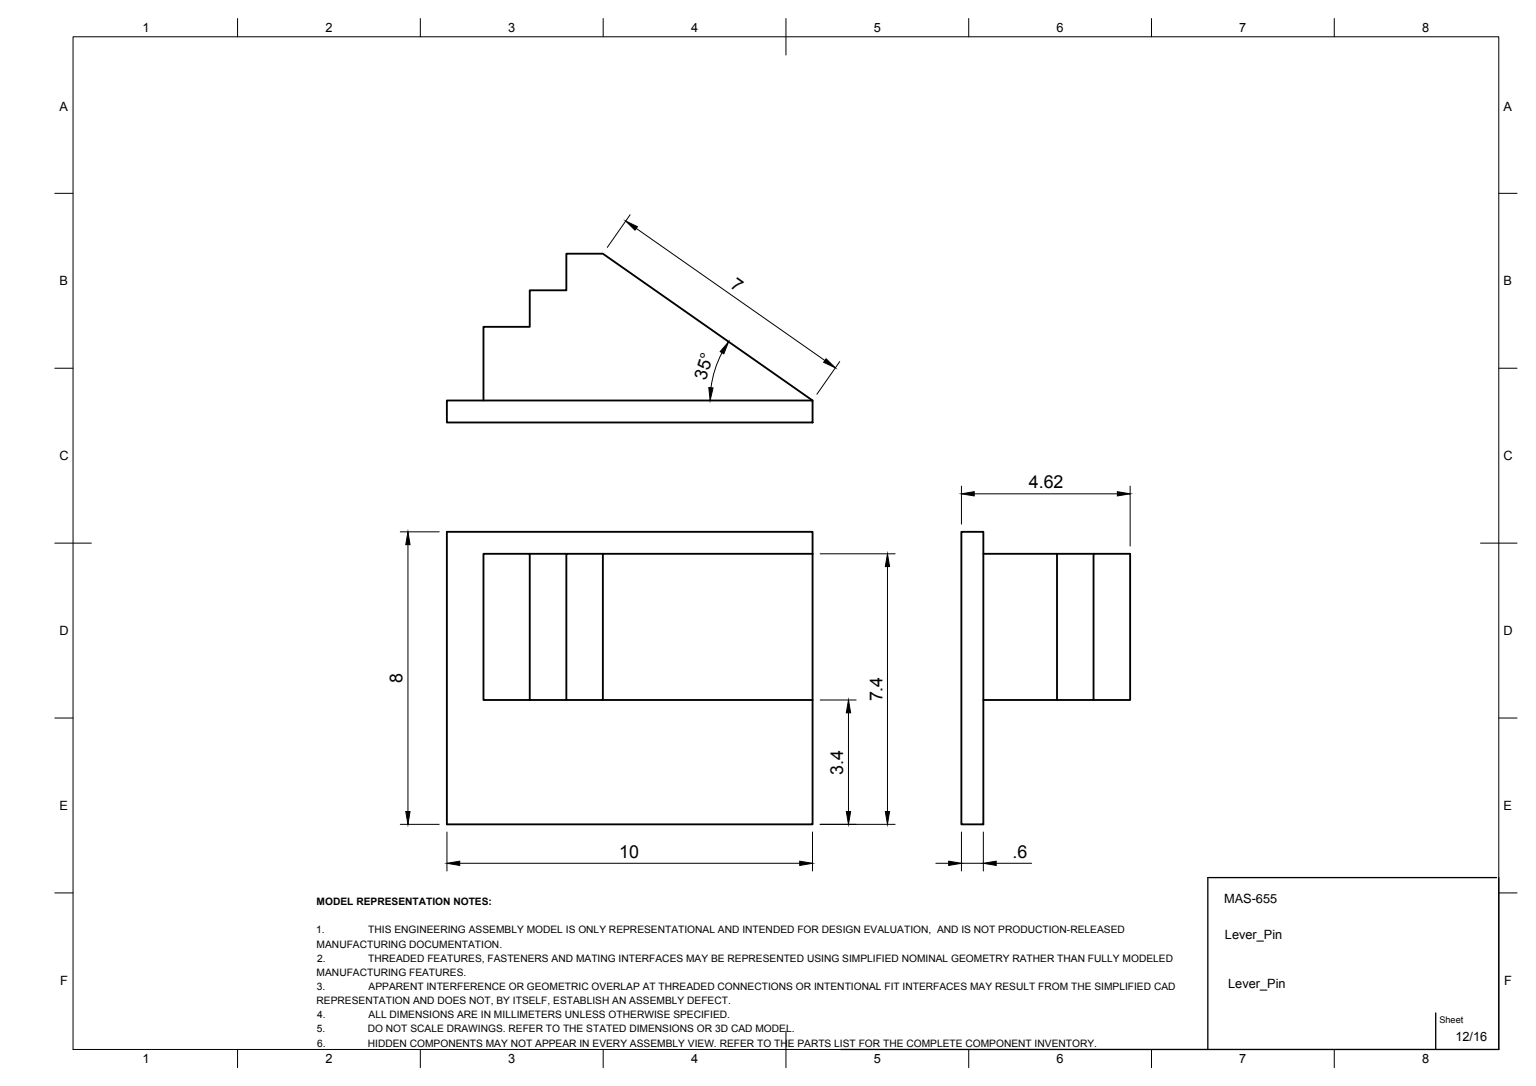
ISO-10303-21;
HEADER;
FILE_DESCRIPTION((''),'2;1');
FILE_NAME('Lever_Pin.step','2026-10-09T11:34:15-07:00',(''),(''),'','','');
FILE_SCHEMA (('AUTOMOTIVE_DESIGN { 1 0 10303 214 3 1 1 }'));
ENDSEC;
DATA;
#10=MECHANICAL_DESIGN_GEOMETRIC_PRESENTATION_REPRESENTATION('',(#644),#117170);
#602=SHAPE_REPRESENTATION_RELATIONSHIP('SRR','None',#117257,#623) ;
#623=ADVANCED_BREP_SHAPE_REPRESENTATION('',(#665),#117165) ;
#644=STYLED_ITEM('',(#117355),#665) ;
#665=MANIFOLD_SOLID_BREP('Body1',#49073) ;
#2840=PLANE('',#54012) ;
#2841=PLANE('',#54013) ;
#2842=PLANE('',#54014) ;
#2843=PLANE('',#54015) ;
#2844=PLANE('',#54016) ;
#2845=PLANE('',#54017) ;
#2846=PLANE('',#54018) ;
#2847=PLANE('',#54019) ;
#2848=PLANE('',#54020) ;
#2849=PLANE('',#54021) ;
#2850=PLANE('',#54022) ;
#2851=PLANE('',#54023) ;
#2852=PLANE('',#54024) ;
#2853=PLANE('',#54025) ;
#2854=PLANE('',#54026) ;
#5713=LINE('',#98676,#8927) ;
#5714=LINE('',#98678,#8928) ;
#5715=LINE('',#98680,#8929) ;
#5716=LINE('',#98681,#8930) ;
#5717=LINE('',#98684,#8931) ;
#5718=LINE('',#98686,#8932) ;
#5719=LINE('',#98687,#8933) ;
#5720=LINE('',#98690,#8934) ;
#5721=LINE('',#98692,#8935) ;
#5722=LINE('',#98693,#8936) ;
#5723=LINE('',#98696,#8937) ;
#5724=LINE('',#98698,#8938) ;
#5725=LINE('',#98699,#8939) ;
#5726=LINE('',#98702,#8940) ;
#5727=LINE('',#98704,#8941) ;
#5728=LINE('',#98705,#8942) ;
#5729=LINE('',#98708,#8943) ;
#5730=LINE('',#98710,#8944) ;
#5731=LINE('',#98711,#8945) ;
#5732=LINE('',#98714,#8946) ;
#5733=LINE('',#98716,#8947) ;
#5734=LINE('',#98717,#8948) ;
#5735=LINE('',#98719,#8949) ;
#5736=LINE('',#98721,#8950) ;
#5737=LINE('',#98725,#8951) ;
#5738=LINE('',#98727,#8952) ;
#5739=LINE('',#98729,#8953) ;
#5740=LINE('',#98730,#8954) ;
#5741=LINE('',#98733,#8955) ;
#5742=LINE('',#98734,#8956) ;
#5743=LINE('',#98736,#8957) ;
#5744=LINE('',#98737,#8958) ;
#5745=LINE('',#98740,#8959) ;
#5746=LINE('',#98742,#8960) ;
#5747=LINE('',#98743,#8961) ;
#5748=LINE('',#98745,#8962) ;
#5749=LINE('',#98746,#8963) ;
#8927=VECTOR('',#67184,10.) ;
#8928=VECTOR('',#67185,10.) ;
#8929=VECTOR('',#67186,10.) ;
#8930=VECTOR('',#67187,10.) ;
#8931=VECTOR('',#67190,10.) ;
#8932=VECTOR('',#67191,10.) ;
#8933=VECTOR('',#67192,10.) ;
#8934=VECTOR('',#67195,10.) ;
#8935=VECTOR('',#67196,10.) ;
#8936=VECTOR('',#67197,10.) ;
#8937=VECTOR('',#67200,10.) ;
#8938=VECTOR('',#67201,10.) ;
#8939=VECTOR('',#67202,10.) ;
#8940=VECTOR('',#67205,10.) ;
#8941=VECTOR('',#67206,10.) ;
#8942=VECTOR('',#67207,10.) ;
#8943=VECTOR('',#67210,10.) ;
#8944=VECTOR('',#67211,10.) ;
#8945=VECTOR('',#67212,10.) ;
#8946=VECTOR('',#67215,10.) ;
#8947=VECTOR('',#67216,10.) ;
#8948=VECTOR('',#67217,10.) ;
#8949=VECTOR('',#67220,10.) ;
#8950=VECTOR('',#67223,10.) ;
#8951=VECTOR('',#67226,10.) ;
#8952=VECTOR('',#67227,10.) ;
#8953=VECTOR('',#67228,10.) ;
#8954=VECTOR('',#67229,10.) ;
#8955=VECTOR('',#67232,10.) ;
#8956=VECTOR('',#67233,10.) ;
#8957=VECTOR('',#67234,10.) ;
#8958=VECTOR('',#67235,10.) ;
#8959=VECTOR('',#67238,10.) ;
#8960=VECTOR('',#67239,10.) ;
#8961=VECTOR('',#67240,10.) ;
#8962=VECTOR('',#67243,10.) ;
#8963=VECTOR('',#67244,10.) ;
#13208=FACE_OUTER_BOUND('',#16391,.T.) ;
#13209=FACE_OUTER_BOUND('',#16392,.T.) ;
#13210=FACE_OUTER_BOUND('',#16393,.T.) ;
#13211=FACE_OUTER_BOUND('',#16394,.T.) ;
#13212=FACE_OUTER_BOUND('',#16395,.T.) ;
#13213=FACE_OUTER_BOUND('',#16396,.T.) ;
#13214=FACE_OUTER_BOUND('',#16397,.T.) ;
#13215=FACE_OUTER_BOUND('',#16398,.T.) ;
#13216=FACE_OUTER_BOUND('',#16399,.T.) ;
#13217=FACE_OUTER_BOUND('',#16400,.T.) ;
#13218=FACE_OUTER_BOUND('',#16401,.T.) ;
#13219=FACE_OUTER_BOUND('',#16402,.T.) ;
#13220=FACE_OUTER_BOUND('',#16403,.T.) ;
#13221=FACE_OUTER_BOUND('',#16404,.T.) ;
#13222=FACE_OUTER_BOUND('',#16405,.T.) ;
#16391=EDGE_LOOP('',(#42608,#42609,#42610,#42611)) ;
#16392=EDGE_LOOP('',(#42612,#42613,#42614,#42615)) ;
#16393=EDGE_LOOP('',(#42616,#42617,#42618,#42619)) ;
#16394=EDGE_LOOP('',(#42620,#42621,#42622,#42623)) ;
#16395=EDGE_LOOP('',(#42624,#42625,#42626,#42627)) ;
#16396=EDGE_LOOP('',(#42628,#42629,#42630,#42631)) ;
#16397=EDGE_LOOP('',(#42632,#42633,#42634,#42635)) ;
#16398=EDGE_LOOP('',(#42636,#42637,#42638,#42639,#42640,#42641,#42642,#42643)) ;
#16399=EDGE_LOOP('',(#42644,#42645,#42646,#42647,#42648,#42649,#42650,#42651)) ;
#16400=EDGE_LOOP('',(#42652,#42653,#42654,#42655)) ;
#16401=EDGE_LOOP('',(#42656,#42657,#42658,#42659,#42660,#42661,#42662,#42663)) ;
#16402=EDGE_LOOP('',(#42664,#42665,#42666,#42667,#42668,#42669)) ;
#16403=EDGE_LOOP('',(#42670,#42671,#42672,#42673)) ;
#16404=EDGE_LOOP('',(#42674,#42675,#42676,#42677)) ;
#16405=EDGE_LOOP('',(#42678,#42679,#42680,#42681)) ;
#22976=VERTEX_POINT('',#98674) ;
#22977=VERTEX_POINT('',#98675) ;
#22978=VERTEX_POINT('',#98677) ;
#22979=VERTEX_POINT('',#98679) ;
#22980=VERTEX_POINT('',#98683) ;
#22981=VERTEX_POINT('',#98685) ;
#22982=VERTEX_POINT('',#98689) ;
#22983=VERTEX_POINT('',#98691) ;
#22984=VERTEX_POINT('',#98695) ;
#22985=VERTEX_POINT('',#98697) ;
#22986=VERTEX_POINT('',#98701) ;
#22987=VERTEX_POINT('',#98703) ;
#22988=VERTEX_POINT('',#98707) ;
#22989=VERTEX_POINT('',#98709) ;
#22990=VERTEX_POINT('',#98713) ;
#22991=VERTEX_POINT('',#98715) ;
#22992=VERTEX_POINT('',#98723) ;
#22993=VERTEX_POINT('',#98724) ;
#22994=VERTEX_POINT('',#98726) ;
#22995=VERTEX_POINT('',#98728) ;
#22996=VERTEX_POINT('',#98732) ;
#22997=VERTEX_POINT('',#98735) ;
#22998=VERTEX_POINT('',#98739) ;
#22999=VERTEX_POINT('',#98741) ;
#29582=EDGE_CURVE('',#22976,#22977,#5713,.T.) ;
#29583=EDGE_CURVE('',#22978,#22977,#5714,.T.) ;
#29584=EDGE_CURVE('',#22979,#22978,#5715,.T.) ;
#29585=EDGE_CURVE('',#22976,#22979,#5716,.T.) ;
#29586=EDGE_CURVE('',#22980,#22976,#5717,.T.) ;
#29587=EDGE_CURVE('',#22981,#22979,#5718,.T.) ;
#29588=EDGE_CURVE('',#22980,#22981,#5719,.T.) ;
#29589=EDGE_CURVE('',#22982,#22980,#5720,.T.) ;
#29590=EDGE_CURVE('',#22983,#22981,#5721,.T.) ;
#29591=EDGE_CURVE('',#22982,#22983,#5722,.T.) ;
#29592=EDGE_CURVE('',#22984,#22982,#5723,.T.) ;
#29593=EDGE_CURVE('',#22985,#22983,#5724,.T.) ;
#29594=EDGE_CURVE('',#22984,#22985,#5725,.T.) ;
#29595=EDGE_CURVE('',#22986,#22984,#5726,.T.) ;
#29596=EDGE_CURVE('',#22987,#22985,#5727,.T.) ;
#29597=EDGE_CURVE('',#22986,#22987,#5728,.T.) ;
#29598=EDGE_CURVE('',#22988,#22986,#5729,.T.) ;
#29599=EDGE_CURVE('',#22989,#22987,#5730,.T.) ;
#29600=EDGE_CURVE('',#22988,#22989,#5731,.T.) ;
#29601=EDGE_CURVE('',#22990,#22988,#5732,.T.) ;
#29602=EDGE_CURVE('',#22991,#22989,#5733,.T.) ;
#29603=EDGE_CURVE('',#22990,#22991,#5734,.T.) ;
#29604=EDGE_CURVE('',#22991,#22978,#5735,.T.) ;
#29605=EDGE_CURVE('',#22977,#22990,#5736,.T.) ;
#29606=EDGE_CURVE('',#22992,#22993,#5737,.T.) ;
#29607=EDGE_CURVE('',#22993,#22994,#5738,.T.) ;
#29608=EDGE_CURVE('',#22995,#22994,#5739,.T.) ;
#29609=EDGE_CURVE('',#22992,#22995,#5740,.T.) ;
#29610=EDGE_CURVE('',#22996,#22990,#5741,.T.) ;
#29611=EDGE_CURVE('',#22996,#22992,#5742,.T.) ;
#29612=EDGE_CURVE('',#22997,#22995,#5743,.T.) ;
#29613=EDGE_CURVE('',#22991,#22997,#5744,.T.) ;
#29614=EDGE_CURVE('',#22998,#22996,#5745,.T.) ;
#29615=EDGE_CURVE('',#22999,#22997,#5746,.T.) ;
#29616=EDGE_CURVE('',#22998,#22999,#5747,.T.) ;
#29617=EDGE_CURVE('',#22993,#22998,#5748,.T.) ;
#29618=EDGE_CURVE('',#22994,#22999,#5749,.T.) ;
#42608=ORIENTED_EDGE('',*,*,#29582,.T.) ;
#42609=ORIENTED_EDGE('',*,*,#29583,.F.) ;
#42610=ORIENTED_EDGE('',*,*,#29584,.F.) ;
#42611=ORIENTED_EDGE('',*,*,#29585,.F.) ;
#42612=ORIENTED_EDGE('',*,*,#29586,.T.) ;
#42613=ORIENTED_EDGE('',*,*,#29585,.T.) ;
#42614=ORIENTED_EDGE('',*,*,#29587,.F.) ;
#42615=ORIENTED_EDGE('',*,*,#29588,.F.) ;
#42616=ORIENTED_EDGE('',*,*,#29589,.T.) ;
#42617=ORIENTED_EDGE('',*,*,#29588,.T.) ;
#42618=ORIENTED_EDGE('',*,*,#29590,.F.) ;
#42619=ORIENTED_EDGE('',*,*,#29591,.F.) ;
#42620=ORIENTED_EDGE('',*,*,#29592,.T.) ;
#42621=ORIENTED_EDGE('',*,*,#29591,.T.) ;
#42622=ORIENTED_EDGE('',*,*,#29593,.F.) ;
#42623=ORIENTED_EDGE('',*,*,#29594,.F.) ;
#42624=ORIENTED_EDGE('',*,*,#29595,.T.) ;
#42625=ORIENTED_EDGE('',*,*,#29594,.T.) ;
#42626=ORIENTED_EDGE('',*,*,#29596,.F.) ;
#42627=ORIENTED_EDGE('',*,*,#29597,.F.) ;
#42628=ORIENTED_EDGE('',*,*,#29598,.T.) ;
#42629=ORIENTED_EDGE('',*,*,#29597,.T.) ;
#42630=ORIENTED_EDGE('',*,*,#29599,.F.) ;
#42631=ORIENTED_EDGE('',*,*,#29600,.F.) ;
#42632=ORIENTED_EDGE('',*,*,#29601,.T.) ;
#42633=ORIENTED_EDGE('',*,*,#29600,.T.) ;
#42634=ORIENTED_EDGE('',*,*,#29602,.F.) ;
#42635=ORIENTED_EDGE('',*,*,#29603,.F.) ;
#42636=ORIENTED_EDGE('',*,*,#29602,.T.) ;
#42637=ORIENTED_EDGE('',*,*,#29599,.T.) ;
#42638=ORIENTED_EDGE('',*,*,#29596,.T.) ;
#42639=ORIENTED_EDGE('',*,*,#29593,.T.) ;
#42640=ORIENTED_EDGE('',*,*,#29590,.T.) ;
#42641=ORIENTED_EDGE('',*,*,#29587,.T.) ;
#42642=ORIENTED_EDGE('',*,*,#29584,.T.) ;
#42643=ORIENTED_EDGE('',*,*,#29604,.F.) ;
#42644=ORIENTED_EDGE('',*,*,#29601,.F.) ;
#42645=ORIENTED_EDGE('',*,*,#29605,.F.) ;
#42646=ORIENTED_EDGE('',*,*,#29582,.F.) ;
#42647=ORIENTED_EDGE('',*,*,#29586,.F.) ;
#42648=ORIENTED_EDGE('',*,*,#29589,.F.) ;
#42649=ORIENTED_EDGE('',*,*,#29592,.F.) ;
#42650=ORIENTED_EDGE('',*,*,#29595,.F.) ;
#42651=ORIENTED_EDGE('',*,*,#29598,.F.) ;
#42652=ORIENTED_EDGE('',*,*,#29606,.T.) ;
#42653=ORIENTED_EDGE('',*,*,#29607,.T.) ;
#42654=ORIENTED_EDGE('',*,*,#29608,.F.) ;
#42655=ORIENTED_EDGE('',*,*,#29609,.F.) ;
#42656=ORIENTED_EDGE('',*,*,#29605,.T.) ;
#42657=ORIENTED_EDGE('',*,*,#29610,.F.) ;
#42658=ORIENTED_EDGE('',*,*,#29611,.T.) ;
#42659=ORIENTED_EDGE('',*,*,#29609,.T.) ;
#42660=ORIENTED_EDGE('',*,*,#29612,.F.) ;
#42661=ORIENTED_EDGE('',*,*,#29613,.F.) ;
#42662=ORIENTED_EDGE('',*,*,#29604,.T.) ;
#42663=ORIENTED_EDGE('',*,*,#29583,.T.) ;
#42664=ORIENTED_EDGE('',*,*,#29614,.T.) ;
#42665=ORIENTED_EDGE('',*,*,#29610,.T.) ;
#42666=ORIENTED_EDGE('',*,*,#29603,.T.) ;
#42667=ORIENTED_EDGE('',*,*,#29613,.T.) ;
#42668=ORIENTED_EDGE('',*,*,#29615,.F.) ;
#42669=ORIENTED_EDGE('',*,*,#29616,.F.) ;
#42670=ORIENTED_EDGE('',*,*,#29617,.T.) ;
#42671=ORIENTED_EDGE('',*,*,#29616,.T.) ;
#42672=ORIENTED_EDGE('',*,*,#29618,.F.) ;
#42673=ORIENTED_EDGE('',*,*,#29607,.F.) ;
#42674=ORIENTED_EDGE('',*,*,#29618,.T.) ;
#42675=ORIENTED_EDGE('',*,*,#29615,.T.) ;
#42676=ORIENTED_EDGE('',*,*,#29612,.T.) ;
#42677=ORIENTED_EDGE('',*,*,#29608,.T.) ;
#42678=ORIENTED_EDGE('',*,*,#29617,.F.) ;
#42679=ORIENTED_EDGE('',*,*,#29606,.F.) ;
#42680=ORIENTED_EDGE('',*,*,#29611,.F.) ;
#42681=ORIENTED_EDGE('',*,*,#29614,.F.) ;
#48426=ADVANCED_FACE('',(#13208),#2840,.T.) ;
#48427=ADVANCED_FACE('',(#13209),#2841,.T.) ;
#48428=ADVANCED_FACE('',(#13210),#2842,.T.) ;
#48429=ADVANCED_FACE('',(#13211),#2843,.T.) ;
#48430=ADVANCED_FACE('',(#13212),#2844,.T.) ;
#48431=ADVANCED_FACE('',(#13213),#2845,.T.) ;
#48432=ADVANCED_FACE('',(#13214),#2846,.T.) ;
#48433=ADVANCED_FACE('',(#13215),#2847,.T.) ;
#48434=ADVANCED_FACE('',(#13216),#2848,.F.) ;
#48435=ADVANCED_FACE('',(#13217),#2849,.T.) ;
#48436=ADVANCED_FACE('',(#13218),#2850,.T.) ;
#48437=ADVANCED_FACE('',(#13219),#2851,.T.) ;
#48438=ADVANCED_FACE('',(#13220),#2852,.T.) ;
#48439=ADVANCED_FACE('',(#13221),#2853,.T.) ;
#48440=ADVANCED_FACE('',(#13222),#2854,.F.) ;
#49073=CLOSED_SHELL('',(#48426,#48427,#48428,#48429,#48430,#48431,#48432,
#48433,#48434,#48435,#48436,#48437,#48438,#48439,#48440)) ;
#54011=AXIS2_PLACEMENT_3D('',#98672,#67180,#67181) ;
#54012=AXIS2_PLACEMENT_3D('',#98673,#67182,#67183) ;
#54013=AXIS2_PLACEMENT_3D('',#98682,#67188,#67189) ;
#54014=AXIS2_PLACEMENT_3D('',#98688,#67193,#67194) ;
#54015=AXIS2_PLACEMENT_3D('',#98694,#67198,#67199) ;
#54016=AXIS2_PLACEMENT_3D('',#98700,#67203,#67204) ;
#54017=AXIS2_PLACEMENT_3D('',#98706,#67208,#67209) ;
#54018=AXIS2_PLACEMENT_3D('',#98712,#67213,#67214) ;
#54019=AXIS2_PLACEMENT_3D('',#98718,#67218,#67219) ;
#54020=AXIS2_PLACEMENT_3D('',#98720,#67221,#67222) ;
#54021=AXIS2_PLACEMENT_3D('',#98722,#67224,#67225) ;
#54022=AXIS2_PLACEMENT_3D('',#98731,#67230,#67231) ;
#54023=AXIS2_PLACEMENT_3D('',#98738,#67236,#67237) ;
#54024=AXIS2_PLACEMENT_3D('',#98744,#67241,#67242) ;
#54025=AXIS2_PLACEMENT_3D('',#98747,#67245,#67246) ;
#54026=AXIS2_PLACEMENT_3D('',#98748,#67247,#67248) ;
#67180=DIRECTION('axis',(0.,0.,1.)) ;
#67181=DIRECTION('refdir',(1.,0.,0.)) ;
#67182=DIRECTION('center_axis',(0.,1.,0.)) ;
#67183=DIRECTION('ref_axis',(1.,0.,0.)) ;
#67184=DIRECTION('',(1.,0.,0.)) ;
#67185=DIRECTION('',(0.,0.,1.)) ;
#67186=DIRECTION('',(1.,0.,0.)) ;
#67187=DIRECTION('',(0.,0.,-1.)) ;
#67188=DIRECTION('center_axis',(-1.,0.,0.)) ;
#67189=DIRECTION('ref_axis',(0.,1.,0.)) ;
#67190=DIRECTION('',(0.,1.,0.)) ;
#67191=DIRECTION('',(0.,1.,0.)) ;
#67192=DIRECTION('',(0.,0.,-1.)) ;
#67193=DIRECTION('center_axis',(0.,1.,0.)) ;
#67194=DIRECTION('ref_axis',(1.,0.,0.)) ;
#67195=DIRECTION('',(1.,0.,0.)) ;
#67196=DIRECTION('',(1.,0.,0.)) ;
#67197=DIRECTION('',(0.,0.,-1.)) ;
#67198=DIRECTION('center_axis',(-1.,0.,0.)) ;
#67199=DIRECTION('ref_axis',(0.,1.,0.)) ;
#67200=DIRECTION('',(0.,1.,0.)) ;
#67201=DIRECTION('',(0.,1.,0.)) ;
#67202=DIRECTION('',(0.,0.,-1.)) ;
#67203=DIRECTION('center_axis',(0.,1.,0.)) ;
#67204=DIRECTION('ref_axis',(1.,0.,0.)) ;
#67205=DIRECTION('',(1.,0.,0.)) ;
#67206=DIRECTION('',(1.,0.,0.)) ;
#67207=DIRECTION('',(0.,0.,-1.)) ;
#67208=DIRECTION('center_axis',(-1.,0.,0.)) ;
#67209=DIRECTION('ref_axis',(0.,1.,0.)) ;
#67210=DIRECTION('',(0.,1.,0.)) ;
#67211=DIRECTION('',(0.,1.,0.)) ;
#67212=DIRECTION('',(0.,0.,-1.)) ;
#67213=DIRECTION('center_axis',(-0.819152044288993,-0.573576436351045,0.)) ;
#67214=DIRECTION('ref_axis',(-0.573576436351045,0.819152044288993,-8.99089246287955E-32)) ;
#67215=DIRECTION('',(-0.573576436351045,0.819152044288993,-8.99089246287955E-32)) ;
#67216=DIRECTION('',(-0.573576436351045,0.819152044288993,-8.99089246287955E-32)) ;
#67217=DIRECTION('',(0.,0.,-1.)) ;
#67218=DIRECTION('center_axis',(0.,0.,-1.)) ;
#67219=DIRECTION('ref_axis',(-1.,0.,0.)) ;
#67220=DIRECTION('',(0.,1.,0.)) ;
#67221=DIRECTION('center_axis',(1.56751426541813E-31,0.,-1.)) ;
#67222=DIRECTION('ref_axis',(1.,0.,1.56751426541813E-31)) ;
#67223=DIRECTION('',(0.,-1.,0.)) ;
#67224=DIRECTION('center_axis',(0.,1.,0.)) ;
#67225=DIRECTION('ref_axis',(1.,0.,0.)) ;
#67226=DIRECTION('',(1.,0.,0.)) ;
#67227=DIRECTION('',(0.,0.,-1.)) ;
#67228=DIRECTION('',(1.,0.,0.)) ;
#67229=DIRECTION('',(0.,0.,-1.)) ;
#67230=DIRECTION('center_axis',(-1.,0.,0.)) ;
#67231=DIRECTION('ref_axis',(0.,1.,0.)) ;
#67232=DIRECTION('',(0.,0.,-1.)) ;
#67233=DIRECTION('',(0.,1.,0.)) ;
#67234=DIRECTION('',(0.,1.,0.)) ;
#67235=DIRECTION('',(0.,0.,-1.)) ;
#67236=DIRECTION('center_axis',(0.,-1.,0.)) ;
#67237=DIRECTION('ref_axis',(-1.,0.,1.04893745400262E-30)) ;
#67238=DIRECTION('',(-1.,0.,1.04893745400262E-30)) ;
#67239=DIRECTION('',(-1.,0.,1.04893745400262E-30)) ;
#67240=DIRECTION('',(0.,0.,-1.)) ;
#67241=DIRECTION('center_axis',(1.,0.,0.)) ;
#67242=DIRECTION('ref_axis',(0.,-1.,-6.29362472401568E-32)) ;
#67243=DIRECTION('',(0.,-1.,-6.29362472401568E-32)) ;
#67244=DIRECTION('',(0.,-1.,-6.29362472401568E-32)) ;
#67245=DIRECTION('center_axis',(0.,0.,-1.)) ;
#67246=DIRECTION('ref_axis',(-1.,0.,0.)) ;
#67247=DIRECTION('center_axis',(-1.04893745400262E-30,0.,-1.)) ;
#67248=DIRECTION('ref_axis',(1.,0.,-1.04893745400262E-30)) ;
#98672=CARTESIAN_POINT('',(0.,0.,0.)) ;
#98673=CARTESIAN_POINT('Origin',(53.3423242584234,235.5,27.7213203435596)) ;
#98674=CARTESIAN_POINT('',(53.3423242584234,235.5,27.7213203435596)) ;
#98675=CARTESIAN_POINT('',(55.3573593128808,235.5,27.7213203435596)) ;
#98676=CARTESIAN_POINT('',(53.3423242584234,235.5,27.7213203435596)) ;
#98677=CARTESIAN_POINT('',(55.3573593128808,235.5,23.7213203435596)) ;
#98678=CARTESIAN_POINT('',(55.3573593128808,235.5,28.0213203435596)) ;
#98679=CARTESIAN_POINT('',(53.3423242584234,235.5,23.7213203435596)) ;
#98680=CARTESIAN_POINT('',(53.3423242584234,235.5,23.7213203435596)) ;
#98681=CARTESIAN_POINT('',(53.3423242584234,235.5,27.7213203435596)) ;
#98682=CARTESIAN_POINT('Origin',(53.3423242584234,234.234064310023,27.7213203435596)) ;
#98683=CARTESIAN_POINT('',(53.3423242584234,234.234064310023,27.7213203435596)) ;
#98684=CARTESIAN_POINT('',(53.3423242584234,234.234064310023,27.7213203435596)) ;
#98685=CARTESIAN_POINT('',(53.3423242584234,234.234064310023,23.7213203435596)) ;
#98686=CARTESIAN_POINT('',(53.3423242584234,234.234064310023,23.7213203435596)) ;
#98687=CARTESIAN_POINT('',(53.3423242584234,234.234064310023,27.7213203435596)) ;
#98688=CARTESIAN_POINT('Origin',(52.3423242584234,234.234064310023,27.7213203435596)) ;
#98689=CARTESIAN_POINT('',(52.3423242584234,234.234064310023,27.7213203435596)) ;
#98690=CARTESIAN_POINT('',(52.3423242584234,234.234064310023,27.7213203435596)) ;
#98691=CARTESIAN_POINT('',(52.3423242584234,234.234064310023,23.7213203435596)) ;
#98692=CARTESIAN_POINT('',(52.3423242584234,234.234064310023,23.7213203435596)) ;
#98693=CARTESIAN_POINT('',(52.3423242584234,234.234064310023,27.7213203435596)) ;
#98694=CARTESIAN_POINT('Origin',(52.3423242584234,233.234064310023,27.7213203435596)) ;
#98695=CARTESIAN_POINT('',(52.3423242584234,233.234064310023,27.7213203435596)) ;
#98696=CARTESIAN_POINT('',(52.3423242584234,233.234064310023,27.7213203435596)) ;
#98697=CARTESIAN_POINT('',(52.3423242584234,233.234064310023,23.7213203435596)) ;
#98698=CARTESIAN_POINT('',(52.3423242584234,233.234064310023,23.7213203435596)) ;
#98699=CARTESIAN_POINT('',(52.3423242584234,233.234064310023,27.7213203435596)) ;
#98700=CARTESIAN_POINT('Origin',(51.3423242584235,233.234064310023,27.7213203435596)) ;
#98701=CARTESIAN_POINT('',(51.3423242584235,233.234064310023,27.7213203435596)) ;
#98702=CARTESIAN_POINT('',(51.3423242584235,233.234064310023,27.7213203435596)) ;
#98703=CARTESIAN_POINT('',(51.3423242584235,233.234064310023,23.7213203435596)) ;
#98704=CARTESIAN_POINT('',(51.3423242584235,233.234064310023,23.7213203435596)) ;
#98705=CARTESIAN_POINT('',(51.3423242584235,233.234064310023,27.7213203435596)) ;
#98706=CARTESIAN_POINT('Origin',(51.3423242584235,232.234064310023,27.7213203435596)) ;
#98707=CARTESIAN_POINT('',(51.3423242584235,232.234064310023,27.7213203435596)) ;
#98708=CARTESIAN_POINT('',(51.3423242584235,232.234064310023,27.7213203435596)) ;
#98709=CARTESIAN_POINT('',(51.3423242584235,232.234064310023,23.7213203435596)) ;
#98710=CARTESIAN_POINT('',(51.3423242584235,232.234064310023,23.7213203435596)) ;
#98711=CARTESIAN_POINT('',(51.3423242584235,232.234064310023,27.7213203435596)) ;
#98712=CARTESIAN_POINT('Origin',(55.3573593128808,226.5,27.7213203435596)) ;
#98713=CARTESIAN_POINT('',(55.3573593128808,226.5,27.7213203435596)) ;
#98714=CARTESIAN_POINT('',(55.3573593128808,226.5,27.7213203435596)) ;
#98715=CARTESIAN_POINT('',(55.3573593128808,226.5,23.7213203435596)) ;
#98716=CARTESIAN_POINT('',(55.3573593128808,226.5,23.7213203435596)) ;
#98717=CARTESIAN_POINT('',(55.3573593128808,226.5,28.3213203435596)) ;
#98718=CARTESIAN_POINT('Origin',(53.3498417856521,231.,23.7213203435596)) ;
#98719=CARTESIAN_POINT('',(55.3573593128808,228.75,23.7213203435596)) ;
#98720=CARTESIAN_POINT('Origin',(53.3498417856521,231.,27.7213203435596)) ;
#98721=CARTESIAN_POINT('',(55.3573593128808,228.75,27.7213203435596)) ;
#98722=CARTESIAN_POINT('Origin',(55.3573593128808,236.5,28.3213203435596)) ;
#98723=CARTESIAN_POINT('',(55.3573593128808,236.5,28.3213203435596)) ;
#98724=CARTESIAN_POINT('',(55.9573593128808,236.5,28.3213203435596)) ;
#98725=CARTESIAN_POINT('',(55.3573593128808,236.5,28.3213203435596)) ;
#98726=CARTESIAN_POINT('',(55.9573593128808,236.5,20.3213203435596)) ;
#98727=CARTESIAN_POINT('',(55.9573593128808,236.5,28.3213203435596)) ;
#98728=CARTESIAN_POINT('',(55.3573593128808,236.5,20.3213203435596)) ;
#98729=CARTESIAN_POINT('',(55.3573593128808,236.5,20.3213203435596)) ;
#98730=CARTESIAN_POINT('',(55.3573593128808,236.5,28.3213203435596)) ;
#98731=CARTESIAN_POINT('Origin',(55.3573593128808,226.5,28.3213203435596)) ;
#98732=CARTESIAN_POINT('',(55.3573593128808,226.5,28.3213203435596)) ;
#98733=CARTESIAN_POINT('',(55.3573593128808,226.5,28.3213203435596)) ;
#98734=CARTESIAN_POINT('',(55.3573593128808,226.5,28.3213203435596)) ;
#98735=CARTESIAN_POINT('',(55.3573593128808,226.5,20.3213203435596)) ;
#98736=CARTESIAN_POINT('',(55.3573593128808,226.5,20.3213203435596)) ;
#98737=CARTESIAN_POINT('',(55.3573593128808,226.5,28.3213203435596)) ;
#98738=CARTESIAN_POINT('Origin',(55.9573593128808,226.5,28.3213203435596)) ;
#98739=CARTESIAN_POINT('',(55.9573593128808,226.5,28.3213203435596)) ;
#98740=CARTESIAN_POINT('',(55.9573593128808,226.5,28.3213203435596)) ;
#98741=CARTESIAN_POINT('',(55.9573593128808,226.5,20.3213203435596)) ;
#98742=CARTESIAN_POINT('',(55.9573593128808,226.5,20.3213203435596)) ;
#98743=CARTESIAN_POINT('',(55.9573593128808,226.5,28.3213203435596)) ;
#98744=CARTESIAN_POINT('Origin',(55.9573593128808,236.5,28.3213203435596)) ;
#98745=CARTESIAN_POINT('',(55.9573593128808,236.5,28.3213203435596)) ;
#98746=CARTESIAN_POINT('',(55.9573593128808,236.5,20.3213203435596)) ;
#98747=CARTESIAN_POINT('Origin',(55.6573593128808,231.5,20.3213203435596)) ;
#98748=CARTESIAN_POINT('Origin',(55.6573593128808,231.5,28.3213203435596)) ;
#117142=UNCERTAINTY_MEASURE_WITH_UNIT(LENGTH_MEASURE(0.01),#117171,
'DISTANCE_ACCURACY_VALUE',
'Maximum model space distance between geometric entities at asserted c
onnectivities') ;
#117147=UNCERTAINTY_MEASURE_WITH_UNIT(LENGTH_MEASURE(0.01),#117171,
'DISTANCE_ACCURACY_VALUE',
'Maximum model space distance between geometric entities at asserted c
onnectivities') ;
#117165=(
GEOMETRIC_REPRESENTATION_CONTEXT(3)
GLOBAL_UNCERTAINTY_ASSIGNED_CONTEXT((#117142))
GLOBAL_UNIT_ASSIGNED_CONTEXT((#117171,#117173,#117174))
REPRESENTATION_CONTEXT('','3D')
) ;
#117170=(
GEOMETRIC_REPRESENTATION_CONTEXT(3)
GLOBAL_UNCERTAINTY_ASSIGNED_CONTEXT((#117147))
GLOBAL_UNIT_ASSIGNED_CONTEXT((#117171,#117173,#117174))
REPRESENTATION_CONTEXT('','3D')
) ;
#117171=(
LENGTH_UNIT()
NAMED_UNIT(*)
SI_UNIT(.MILLI.,.METRE.)
) ;
#117173=(
NAMED_UNIT(*)
PLANE_ANGLE_UNIT()
SI_UNIT($,.RADIAN.)
) ;
#117174=(
NAMED_UNIT(*)
SI_UNIT($,.STERADIAN.)
SOLID_ANGLE_UNIT()
) ;
#117192=SHAPE_DEFINITION_REPRESENTATION(#117214,#117257) ;
#117214=PRODUCT_DEFINITION_SHAPE('',$,#117280) ;
#117257=SHAPE_REPRESENTATION('',(#54011),#117165) ;
#117262=PRODUCT_DEFINITION_CONTEXT('part definition',#117330,'design') ;
#117280=PRODUCT_DEFINITION('Lever_Pin','Lever_Pin',#117302,#117262) ;
#117302=PRODUCT_DEFINITION_FORMATION('',$,#117349) ;
#117330=APPLICATION_CONTEXT(
'Core Data for Automotive Mechanical Design Process') ;
#117331=PRODUCT_CONTEXT('part definition',#117330,'mechanical') ;
#117349=PRODUCT('Lever_Pin','Lever_Pin',$,(#117331)) ;
#117355=PRESENTATION_STYLE_ASSIGNMENT((#117357)) ;
#117357=SURFACE_STYLE_USAGE(.BOTH.,#117359) ;
#117359=SURFACE_SIDE_STYLE('',(#117361)) ;
#117361=SURFACE_STYLE_FILL_AREA(#117363) ;
#117363=FILL_AREA_STYLE('Opaque(160,160,160)',(#117365)) ;
#117365=FILL_AREA_STYLE_COLOUR('Opaque(160,160,160)',#117367) ;
#117367=COLOUR_RGB('Opaque(160,160,160)', 0.09019608, 0.27058824, 0.51372549) ;
ENDSEC;
END-ISO-10303-21;
